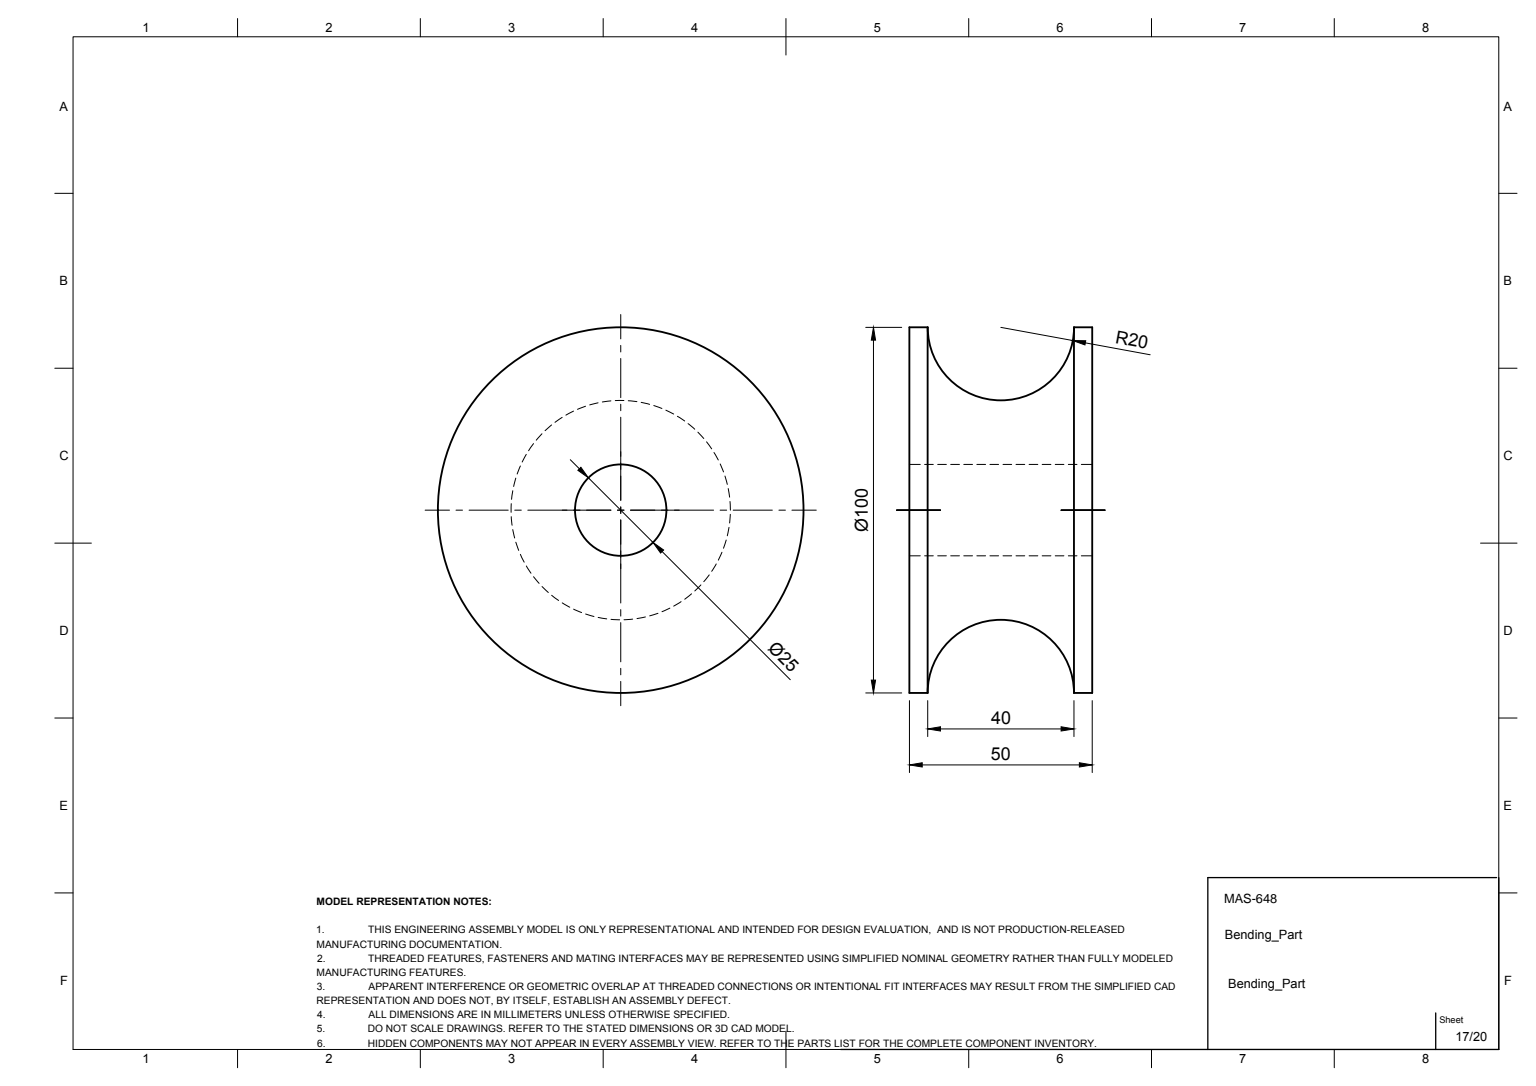
ISO-10303-21;
HEADER;
FILE_DESCRIPTION((''),'2;1');
FILE_NAME('Bending_Part.step','2026-10-09T12:47:58-07:00',(''),(''),'','','');
FILE_SCHEMA (('AUTOMOTIVE_DESIGN { 1 0 10303 214 3 1 1 }'));
ENDSEC;
DATA;
#10=MECHANICAL_DESIGN_GEOMETRIC_PRESENTATION_REPRESENTATION('',(#318),#3475);
#23=TOROIDAL_SURFACE('',#2087,50.,20.) ;
#157=FACE_BOUND('',#532,.T.) ;
#158=FACE_BOUND('',#534,.T.) ;
#198=CIRCLE('',#2088,50.) ;
#199=CIRCLE('',#2089,20.) ;
#200=CIRCLE('',#2090,50.) ;
#201=CIRCLE('',#2091,50.) ;
#202=CIRCLE('',#2092,50.) ;
#203=CIRCLE('',#2094,12.5) ;
#204=CIRCLE('',#2095,12.5) ;
#205=CIRCLE('',#2097,50.) ;
#206=CIRCLE('',#2099,50.) ;
#273=CYLINDRICAL_SURFACE('',#2093,12.5) ;
#274=CYLINDRICAL_SURFACE('',#2096,50.) ;
#275=CYLINDRICAL_SURFACE('',#2098,50.) ;
#294=SHAPE_REPRESENTATION_RELATIONSHIP('SRR','None',#3550,#306) ;
#306=ADVANCED_BREP_SHAPE_REPRESENTATION('',(#330),#3470) ;
#318=STYLED_ITEM('',(#3628),#330) ;
#330=MANIFOLD_SOLID_BREP('Body1',#1832) ;
#397=FACE_OUTER_BOUND('',#527,.T.) ;
#398=FACE_OUTER_BOUND('',#528,.T.) ;
#399=FACE_OUTER_BOUND('',#529,.T.) ;
#400=FACE_OUTER_BOUND('',#530,.T.) ;
#401=FACE_OUTER_BOUND('',#531,.T.) ;
#402=FACE_OUTER_BOUND('',#533,.T.) ;
#527=EDGE_LOOP('',(#1440,#1441,#1442,#1443,#1444,#1445)) ;
#528=EDGE_LOOP('',(#1446,#1447,#1448,#1449)) ;
#529=EDGE_LOOP('',(#1450,#1451,#1452,#1453,#1454)) ;
#530=EDGE_LOOP('',(#1455,#1456,#1457,#1458,#1459)) ;
#531=EDGE_LOOP('',(#1460)) ;
#532=EDGE_LOOP('',(#1461)) ;
#533=EDGE_LOOP('',(#1462)) ;
#534=EDGE_LOOP('',(#1463)) ;
#674=LINE('',#3197,#793) ;
#675=LINE('',#3202,#794) ;
#676=LINE('',#3205,#795) ;
#793=VECTOR('',#2553,12.5) ;
#794=VECTOR('',#2560,50.) ;
#795=VECTOR('',#2563,50.) ;
#907=VERTEX_POINT('',#3184) ;
#908=VERTEX_POINT('',#3185) ;
#909=VERTEX_POINT('',#3187) ;
#910=VERTEX_POINT('',#3189) ;
#911=VERTEX_POINT('',#3194) ;
#912=VERTEX_POINT('',#3196) ;
#913=VERTEX_POINT('',#3200) ;
#914=VERTEX_POINT('',#3204) ;
#1092=EDGE_CURVE('',#907,#908,#198,.T.) ;
#1093=EDGE_CURVE('',#908,#909,#199,.T.) ;
#1094=EDGE_CURVE('',#909,#910,#200,.T.) ;
#1095=EDGE_CURVE('',#910,#909,#201,.T.) ;
#1096=EDGE_CURVE('',#908,#907,#202,.T.) ;
#1097=EDGE_CURVE('',#911,#911,#203,.T.) ;
#1098=EDGE_CURVE('',#911,#912,#674,.T.) ;
#1099=EDGE_CURVE('',#912,#912,#204,.T.) ;
#1100=EDGE_CURVE('',#913,#913,#205,.T.) ;
#1101=EDGE_CURVE('',#913,#910,#675,.T.) ;
#1102=EDGE_CURVE('',#907,#914,#676,.T.) ;
#1103=EDGE_CURVE('',#914,#914,#206,.T.) ;
#1440=ORIENTED_EDGE('',*,*,#1092,.T.) ;
#1441=ORIENTED_EDGE('',*,*,#1093,.T.) ;
#1442=ORIENTED_EDGE('',*,*,#1094,.T.) ;
#1443=ORIENTED_EDGE('',*,*,#1095,.T.) ;
#1444=ORIENTED_EDGE('',*,*,#1093,.F.) ;
#1445=ORIENTED_EDGE('',*,*,#1096,.T.) ;
#1446=ORIENTED_EDGE('',*,*,#1097,.F.) ;
#1447=ORIENTED_EDGE('',*,*,#1098,.T.) ;
#1448=ORIENTED_EDGE('',*,*,#1099,.T.) ;
#1449=ORIENTED_EDGE('',*,*,#1098,.F.) ;
#1450=ORIENTED_EDGE('',*,*,#1100,.T.) ;
#1451=ORIENTED_EDGE('',*,*,#1101,.T.) ;
#1452=ORIENTED_EDGE('',*,*,#1094,.F.) ;
#1453=ORIENTED_EDGE('',*,*,#1095,.F.) ;
#1454=ORIENTED_EDGE('',*,*,#1101,.F.) ;
#1455=ORIENTED_EDGE('',*,*,#1092,.F.) ;
#1456=ORIENTED_EDGE('',*,*,#1102,.T.) ;
#1457=ORIENTED_EDGE('',*,*,#1103,.F.) ;
#1458=ORIENTED_EDGE('',*,*,#1102,.F.) ;
#1459=ORIENTED_EDGE('',*,*,#1096,.F.) ;
#1460=ORIENTED_EDGE('',*,*,#1103,.T.) ;
#1461=ORIENTED_EDGE('',*,*,#1099,.F.) ;
#1462=ORIENTED_EDGE('',*,*,#1100,.F.) ;
#1463=ORIENTED_EDGE('',*,*,#1097,.T.) ;
#1687=PLANE('',#2100) ;
#1688=PLANE('',#2101) ;
#1773=ADVANCED_FACE('',(#397),#23,.F.) ;
#1774=ADVANCED_FACE('',(#398),#273,.F.) ;
#1775=ADVANCED_FACE('',(#399),#274,.T.) ;
#1776=ADVANCED_FACE('',(#400),#275,.T.) ;
#1777=ADVANCED_FACE('',(#401,#157),#1687,.T.) ;
#1778=ADVANCED_FACE('',(#402,#158),#1688,.F.) ;
#1832=CLOSED_SHELL('',(#1773,#1774,#1775,#1776,#1777,#1778)) ;
#2086=AXIS2_PLACEMENT_3D('',#3182,#2535,#2536) ;
#2087=AXIS2_PLACEMENT_3D('',#3183,#2537,#2538) ;
#2088=AXIS2_PLACEMENT_3D('',#3186,#2539,#2540) ;
#2089=AXIS2_PLACEMENT_3D('',#3188,#2541,#2542) ;
#2090=AXIS2_PLACEMENT_3D('',#3190,#2543,#2544) ;
#2091=AXIS2_PLACEMENT_3D('',#3191,#2545,#2546) ;
#2092=AXIS2_PLACEMENT_3D('',#3192,#2547,#2548) ;
#2093=AXIS2_PLACEMENT_3D('',#3193,#2549,#2550) ;
#2094=AXIS2_PLACEMENT_3D('',#3195,#2551,#2552) ;
#2095=AXIS2_PLACEMENT_3D('',#3198,#2554,#2555) ;
#2096=AXIS2_PLACEMENT_3D('',#3199,#2556,#2557) ;
#2097=AXIS2_PLACEMENT_3D('',#3201,#2558,#2559) ;
#2098=AXIS2_PLACEMENT_3D('',#3203,#2561,#2562) ;
#2099=AXIS2_PLACEMENT_3D('',#3206,#2564,#2565) ;
#2100=AXIS2_PLACEMENT_3D('',#3207,#2566,#2567) ;
#2101=AXIS2_PLACEMENT_3D('',#3208,#2568,#2569) ;
#2535=DIRECTION('axis',(0.,0.,1.)) ;
#2536=DIRECTION('refdir',(1.,0.,0.)) ;
#2537=DIRECTION('center_axis',(0.,0.,1.)) ;
#2538=DIRECTION('ref_axis',(1.,0.,0.)) ;
#2539=DIRECTION('center_axis',(0.,0.,-1.)) ;
#2540=DIRECTION('ref_axis',(-1.,0.,0.)) ;
#2541=DIRECTION('center_axis',(-1.22464679914735E-16,1.,0.)) ;
#2542=DIRECTION('ref_axis',(-1.,-1.22464679914735E-16,0.)) ;
#2543=DIRECTION('center_axis',(0.,0.,1.)) ;
#2544=DIRECTION('ref_axis',(1.,0.,0.)) ;
#2545=DIRECTION('center_axis',(0.,0.,1.)) ;
#2546=DIRECTION('ref_axis',(1.,0.,0.)) ;
#2547=DIRECTION('center_axis',(0.,0.,-1.)) ;
#2548=DIRECTION('ref_axis',(-1.,0.,0.)) ;
#2549=DIRECTION('center_axis',(0.,0.,1.)) ;
#2550=DIRECTION('ref_axis',(1.,0.,0.)) ;
#2551=DIRECTION('center_axis',(0.,0.,1.)) ;
#2552=DIRECTION('ref_axis',(1.,0.,0.)) ;
#2553=DIRECTION('',(0.,0.,1.)) ;
#2554=DIRECTION('center_axis',(0.,0.,1.)) ;
#2555=DIRECTION('ref_axis',(1.,0.,0.)) ;
#2556=DIRECTION('center_axis',(0.,0.,-1.)) ;
#2557=DIRECTION('ref_axis',(-1.,0.,0.)) ;
#2558=DIRECTION('center_axis',(0.,0.,1.)) ;
#2559=DIRECTION('ref_axis',(1.,0.,0.)) ;
#2560=DIRECTION('',(0.,0.,1.)) ;
#2561=DIRECTION('center_axis',(0.,0.,-1.)) ;
#2562=DIRECTION('ref_axis',(-1.,0.,0.)) ;
#2563=DIRECTION('',(0.,0.,1.)) ;
#2564=DIRECTION('center_axis',(0.,0.,1.)) ;
#2565=DIRECTION('ref_axis',(1.,0.,0.)) ;
#2566=DIRECTION('center_axis',(0.,0.,1.)) ;
#2567=DIRECTION('ref_axis',(1.,0.,0.)) ;
#2568=DIRECTION('center_axis',(0.,0.,1.)) ;
#2569=DIRECTION('ref_axis',(1.,0.,0.)) ;
#3182=CARTESIAN_POINT('',(0.,0.,0.)) ;
#3183=CARTESIAN_POINT('Origin',(0.,0.,0.)) ;
#3184=CARTESIAN_POINT('',(50.,-6.12323399573677E-15,20.)) ;
#3185=CARTESIAN_POINT('',(-50.,-6.12323399573677E-15,20.)) ;
#3186=CARTESIAN_POINT('Origin',(0.,0.,20.)) ;
#3187=CARTESIAN_POINT('',(-50.,-6.12323399573677E-15,-20.)) ;
#3188=CARTESIAN_POINT('Origin',(-50.,-6.12323399573677E-15,0.)) ;
#3189=CARTESIAN_POINT('',(50.,-6.12323399573677E-15,-20.)) ;
#3190=CARTESIAN_POINT('Origin',(0.,0.,-20.)) ;
#3191=CARTESIAN_POINT('Origin',(0.,0.,-20.)) ;
#3192=CARTESIAN_POINT('Origin',(0.,0.,20.)) ;
#3193=CARTESIAN_POINT('Origin',(0.,0.,-25.)) ;
#3194=CARTESIAN_POINT('',(-12.5,-1.53080849893419E-15,-25.)) ;
#3195=CARTESIAN_POINT('Origin',(0.,0.,-25.)) ;
#3196=CARTESIAN_POINT('',(-12.5,-1.53080849893419E-15,25.)) ;
#3197=CARTESIAN_POINT('',(-12.5,-1.53080849893419E-15,-25.)) ;
#3198=CARTESIAN_POINT('Origin',(0.,0.,25.)) ;
#3199=CARTESIAN_POINT('Origin',(0.,0.,25.)) ;
#3200=CARTESIAN_POINT('',(50.,-6.12323399573677E-15,-25.)) ;
#3201=CARTESIAN_POINT('Origin',(0.,0.,-25.)) ;
#3202=CARTESIAN_POINT('',(50.,-6.12323399573677E-15,25.)) ;
#3203=CARTESIAN_POINT('Origin',(0.,0.,25.)) ;
#3204=CARTESIAN_POINT('',(50.,-6.12323399573677E-15,25.)) ;
#3205=CARTESIAN_POINT('',(50.,-6.12323399573677E-15,25.)) ;
#3206=CARTESIAN_POINT('Origin',(0.,0.,25.)) ;
#3207=CARTESIAN_POINT('Origin',(0.,0.,25.)) ;
#3208=CARTESIAN_POINT('Origin',(0.,0.,-25.)) ;
#3452=UNCERTAINTY_MEASURE_WITH_UNIT(LENGTH_MEASURE(0.01),#3476,
'DISTANCE_ACCURACY_VALUE',
'Maximum model space distance between geometric entities at asserted c
onnectivities') ;
#3457=UNCERTAINTY_MEASURE_WITH_UNIT(LENGTH_MEASURE(0.01),#3476,
'DISTANCE_ACCURACY_VALUE',
'Maximum model space distance between geometric entities at asserted c
onnectivities') ;
#3470=(
GEOMETRIC_REPRESENTATION_CONTEXT(3)
GLOBAL_UNCERTAINTY_ASSIGNED_CONTEXT((#3452))
GLOBAL_UNIT_ASSIGNED_CONTEXT((#3476,#3478,#3479))
REPRESENTATION_CONTEXT('','3D')
) ;
#3475=(
GEOMETRIC_REPRESENTATION_CONTEXT(3)
GLOBAL_UNCERTAINTY_ASSIGNED_CONTEXT((#3457))
GLOBAL_UNIT_ASSIGNED_CONTEXT((#3476,#3478,#3479))
REPRESENTATION_CONTEXT('','3D')
) ;
#3476=(
LENGTH_UNIT()
NAMED_UNIT(*)
SI_UNIT(.MILLI.,.METRE.)
) ;
#3478=(
NAMED_UNIT(*)
PLANE_ANGLE_UNIT()
SI_UNIT($,.RADIAN.)
) ;
#3479=(
NAMED_UNIT(*)
SI_UNIT($,.STERADIAN.)
SOLID_ANGLE_UNIT()
) ;
#3492=SHAPE_DEFINITION_REPRESENTATION(#3519,#3550) ;
#3519=PRODUCT_DEFINITION_SHAPE('',$,#3568) ;
#3550=SHAPE_REPRESENTATION('',(#2086),#3470) ;
#3555=PRODUCT_DEFINITION_CONTEXT('part definition',#3608,'design') ;
#3568=PRODUCT_DEFINITION('Bending_Part',
'Bending_Part',#3585,#3555) ;
#3585=PRODUCT_DEFINITION_FORMATION('',$,#3622) ;
#3608=APPLICATION_CONTEXT(
'Core Data for Automotive Mechanical Design Process') ;
#3609=PRODUCT_CONTEXT('part definition',#3608,'mechanical') ;
#3622=PRODUCT('Bending_Part','Bending_Part',$,
(#3609)) ;
#3628=PRESENTATION_STYLE_ASSIGNMENT((#3630)) ;
#3630=SURFACE_STYLE_USAGE(.BOTH.,#3632) ;
#3632=SURFACE_SIDE_STYLE('',(#3634)) ;
#3634=SURFACE_STYLE_FILL_AREA(#3636) ;
#3636=FILL_AREA_STYLE('Opaque(202,209,238)',(#3638)) ;
#3638=FILL_AREA_STYLE_COLOUR('Opaque(202,209,238)',#3640) ;
#3640=COLOUR_RGB('Opaque(202,209,238)', 0.09019608, 0.27058824, 0.51372549) ;
ENDSEC;
END-ISO-10303-21;
